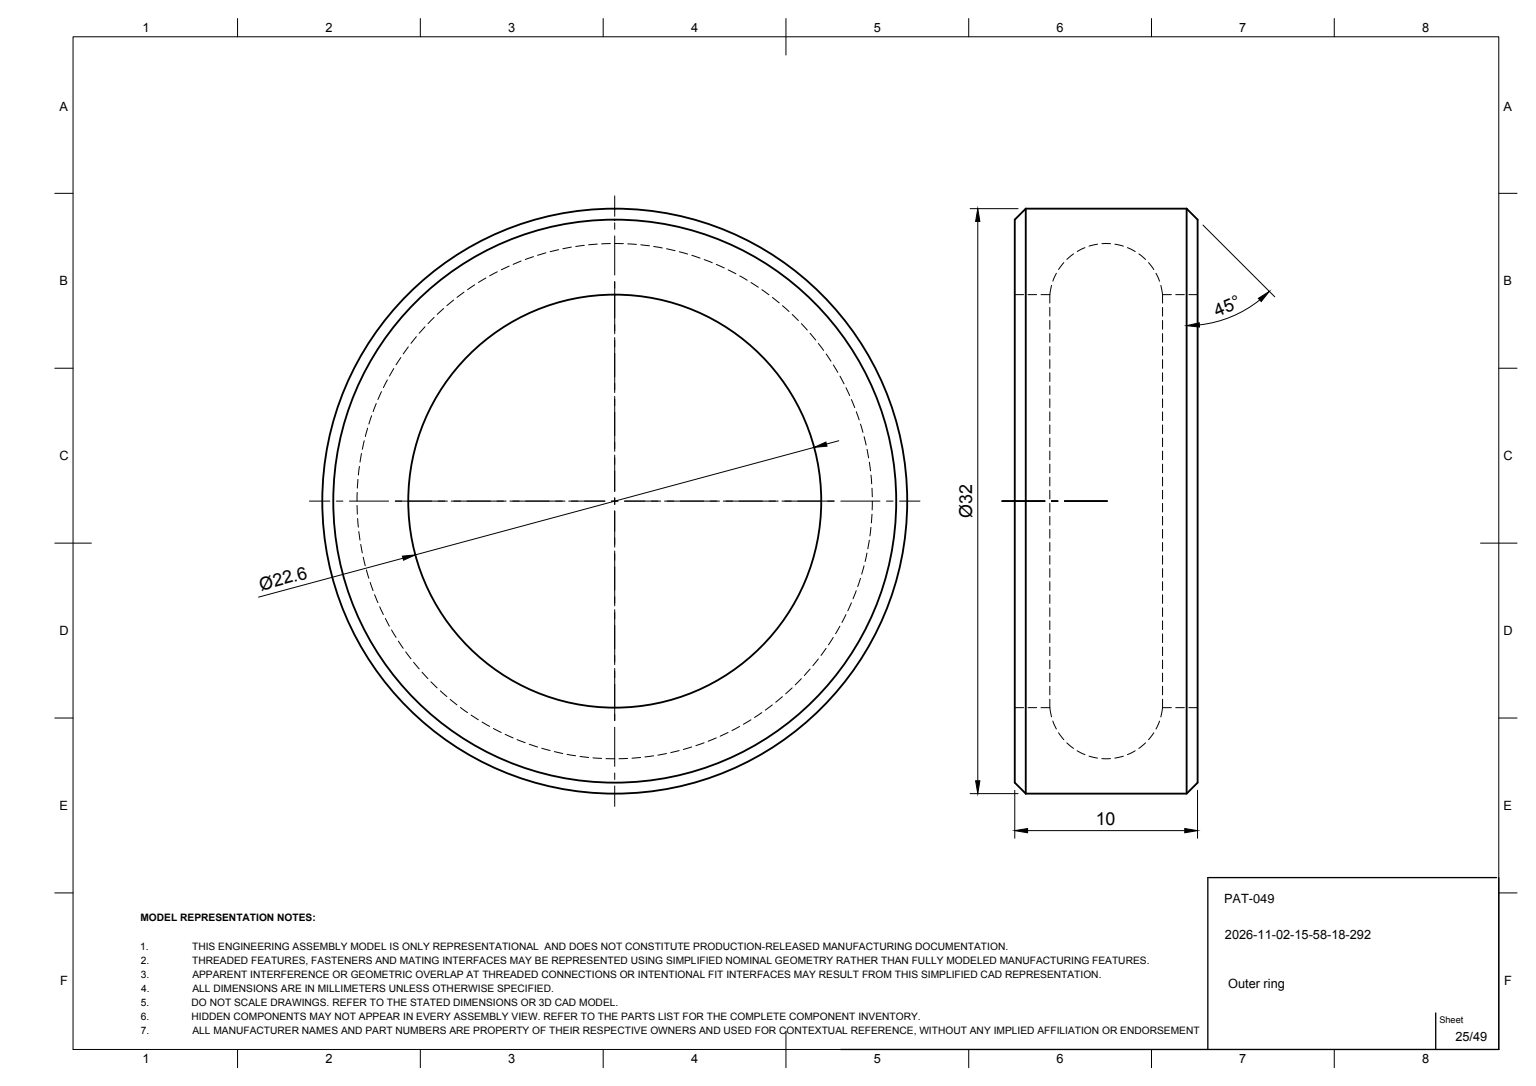
ISO-10303-21;
HEADER;
/* Generated by software containing ST-Developer
 * from STEP Tools, Inc. (www.steptools.com) 
 */

FILE_DESCRIPTION(
/* description */ ('Hand drill press frame (manual)'),
/* implementation_level */ '2;1');

FILE_NAME(
/* name */ 'Outer ring.step',
/* time_stamp */ '2026-10-28T03:25:28-07:00',
/* author */ (''),
/* organization */ (''),
/* preprocessor_version */ 'ST-DEVELOPER v20.2',
/* originating_system */ 'Autodesk Translation Framework v15.17.0.0',
/* authorisation */ '');

FILE_SCHEMA (('AUTOMOTIVE_DESIGN { 1 0 10303 214 3 1 1 }'));
ENDSEC;

DATA;
#10=MECHANICAL_DESIGN_GEOMETRIC_PRESENTATION_REPRESENTATION('',(#637),#33299);
#472=TOROIDAL_SURFACE('',#13625,1.1,0.309556);
#476=CONICAL_SURFACE('',#13636,1.57,0.785398163397449);
#477=CONICAL_SURFACE('',#13640,1.57,0.785398163397449);
#547=SHAPE_REPRESENTATION_RELATIONSHIP('SRR','None',#33507,#592);
#592=ADVANCED_BREP_SHAPE_REPRESENTATION('',(#689),#33269);
#637=STYLED_ITEM('',(#33814),#689);
#689=MANIFOLD_SOLID_BREP('Body1',#12655);
#838=FACE_BOUND('',#2374,.T.);
#839=FACE_BOUND('',#2379,.T.);
#1019=PLANE('',#13633);
#1020=PLANE('',#13642);
#1564=FACE_OUTER_BOUND('',#2371,.T.);
#1565=FACE_OUTER_BOUND('',#2372,.T.);
#1566=FACE_OUTER_BOUND('',#2373,.T.);
#1567=FACE_OUTER_BOUND('',#2375,.T.);
#1568=FACE_OUTER_BOUND('',#2376,.T.);
#1569=FACE_OUTER_BOUND('',#2377,.T.);
#1570=FACE_OUTER_BOUND('',#2378,.T.);
#1571=FACE_OUTER_BOUND('',#2380,.T.);
#2371=EDGE_LOOP('',(#9479,#9480,#9481,#9482,#9483,#9484));
#2372=EDGE_LOOP('',(#9485,#9486,#9487,#9488,#9489));
#2373=EDGE_LOOP('',(#9490));
#2374=EDGE_LOOP('',(#9491));
#2375=EDGE_LOOP('',(#9492,#9493,#9494,#9495));
#2376=EDGE_LOOP('',(#9496,#9497,#9498,#9499));
#2377=EDGE_LOOP('',(#9500,#9501,#9502,#9503));
#2378=EDGE_LOOP('',(#9504));
#2379=EDGE_LOOP('',(#9505));
#2380=EDGE_LOOP('',(#9506,#9507,#9508,#9509,#9510));
#3208=LINE('',#19214,#4373);
#3209=LINE('',#19223,#4374);
#3210=LINE('',#19227,#4375);
#3211=LINE('',#19231,#4376);
#3212=LINE('',#19234,#4377);
#4373=VECTOR('',#15581,1.129765);
#4374=VECTOR('',#15592,1.57);
#4375=VECTOR('',#15597,1.6);
#4376=VECTOR('',#15602,1.57);
#4377=VECTOR('',#15607,1.129765);
#5404=CIRCLE('',#13626,1.129765);
#5405=CIRCLE('',#13627,1.129765);
#5406=CIRCLE('',#13628,0.309556);
#5407=CIRCLE('',#13629,1.129765);
#5408=CIRCLE('',#13630,1.129765);
#5409=CIRCLE('',#13632,1.129765);
#5410=CIRCLE('',#13634,1.54);
#5411=CIRCLE('',#13635,1.129765);
#5412=CIRCLE('',#13637,1.6);
#5413=CIRCLE('',#13639,1.6);
#5414=CIRCLE('',#13641,1.54);
#5965=VERTEX_POINT('',#19202);
#5966=VERTEX_POINT('',#19203);
#5967=VERTEX_POINT('',#19206);
#5968=VERTEX_POINT('',#19208);
#5969=VERTEX_POINT('',#19212);
#5970=VERTEX_POINT('',#19216);
#5971=VERTEX_POINT('',#19218);
#5972=VERTEX_POINT('',#19221);
#5973=VERTEX_POINT('',#19225);
#5974=VERTEX_POINT('',#19229);
#7268=EDGE_CURVE('',#5965,#5966,#5404,.T.);
#7269=EDGE_CURVE('',#5966,#5965,#5405,.T.);
#7270=EDGE_CURVE('',#5966,#5967,#5406,.T.);
#7271=EDGE_CURVE('',#5968,#5967,#5407,.T.);
#7272=EDGE_CURVE('',#5967,#5968,#5408,.T.);
#7273=EDGE_CURVE('',#5969,#5969,#5409,.T.);
#7274=EDGE_CURVE('',#5969,#5968,#3208,.T.);
#7275=EDGE_CURVE('',#5970,#5970,#5410,.T.);
#7276=EDGE_CURVE('',#5971,#5971,#5411,.T.);
#7277=EDGE_CURVE('',#5972,#5972,#5412,.T.);
#7278=EDGE_CURVE('',#5972,#5970,#3209,.T.);
#7279=EDGE_CURVE('',#5973,#5973,#5413,.T.);
#7280=EDGE_CURVE('',#5973,#5972,#3210,.T.);
#7281=EDGE_CURVE('',#5974,#5974,#5414,.T.);
#7282=EDGE_CURVE('',#5974,#5973,#3211,.T.);
#7283=EDGE_CURVE('',#5965,#5971,#3212,.T.);
#9479=ORIENTED_EDGE('',*,*,#7268,.F.);
#9480=ORIENTED_EDGE('',*,*,#7269,.F.);
#9481=ORIENTED_EDGE('',*,*,#7270,.T.);
#9482=ORIENTED_EDGE('',*,*,#7271,.F.);
#9483=ORIENTED_EDGE('',*,*,#7272,.F.);
#9484=ORIENTED_EDGE('',*,*,#7270,.F.);
#9485=ORIENTED_EDGE('',*,*,#7273,.T.);
#9486=ORIENTED_EDGE('',*,*,#7274,.T.);
#9487=ORIENTED_EDGE('',*,*,#7271,.T.);
#9488=ORIENTED_EDGE('',*,*,#7272,.T.);
#9489=ORIENTED_EDGE('',*,*,#7274,.F.);
#9490=ORIENTED_EDGE('',*,*,#7275,.F.);
#9491=ORIENTED_EDGE('',*,*,#7276,.T.);
#9492=ORIENTED_EDGE('',*,*,#7277,.F.);
#9493=ORIENTED_EDGE('',*,*,#7278,.T.);
#9494=ORIENTED_EDGE('',*,*,#7275,.T.);
#9495=ORIENTED_EDGE('',*,*,#7278,.F.);
#9496=ORIENTED_EDGE('',*,*,#7279,.F.);
#9497=ORIENTED_EDGE('',*,*,#7280,.T.);
#9498=ORIENTED_EDGE('',*,*,#7277,.T.);
#9499=ORIENTED_EDGE('',*,*,#7280,.F.);
#9500=ORIENTED_EDGE('',*,*,#7281,.F.);
#9501=ORIENTED_EDGE('',*,*,#7282,.T.);
#9502=ORIENTED_EDGE('',*,*,#7279,.T.);
#9503=ORIENTED_EDGE('',*,*,#7282,.F.);
#9504=ORIENTED_EDGE('',*,*,#7281,.T.);
#9505=ORIENTED_EDGE('',*,*,#7273,.F.);
#9506=ORIENTED_EDGE('',*,*,#7268,.T.);
#9507=ORIENTED_EDGE('',*,*,#7269,.T.);
#9508=ORIENTED_EDGE('',*,*,#7283,.T.);
#9509=ORIENTED_EDGE('',*,*,#7276,.F.);
#9510=ORIENTED_EDGE('',*,*,#7283,.F.);
#11874=CYLINDRICAL_SURFACE('',#13631,1.129765);
#11875=CYLINDRICAL_SURFACE('',#13638,1.6);
#11876=CYLINDRICAL_SURFACE('',#13643,1.129765);
#12173=ADVANCED_FACE('',(#1564),#472,.F.);
#12174=ADVANCED_FACE('',(#1565),#11874,.F.);
#12175=ADVANCED_FACE('',(#1566,#838),#1019,.T.);
#12176=ADVANCED_FACE('',(#1567),#476,.T.);
#12177=ADVANCED_FACE('',(#1568),#11875,.T.);
#12178=ADVANCED_FACE('',(#1569),#477,.T.);
#12179=ADVANCED_FACE('',(#1570,#839),#1020,.T.);
#12180=ADVANCED_FACE('',(#1571),#11876,.F.);
#12655=CLOSED_SHELL('',(#12173,#12174,#12175,#12176,#12177,#12178,#12179,
#12180));
#13624=AXIS2_PLACEMENT_3D('',#19200,#15563,#15564);
#13625=AXIS2_PLACEMENT_3D('',#19201,#15565,#15566);
#13626=AXIS2_PLACEMENT_3D('',#19204,#15567,#15568);
#13627=AXIS2_PLACEMENT_3D('',#19205,#15569,#15570);
#13628=AXIS2_PLACEMENT_3D('',#19207,#15571,#15572);
#13629=AXIS2_PLACEMENT_3D('',#19209,#15573,#15574);
#13630=AXIS2_PLACEMENT_3D('',#19210,#15575,#15576);
#13631=AXIS2_PLACEMENT_3D('',#19211,#15577,#15578);
#13632=AXIS2_PLACEMENT_3D('',#19213,#15579,#15580);
#13633=AXIS2_PLACEMENT_3D('',#19215,#15582,#15583);
#13634=AXIS2_PLACEMENT_3D('',#19217,#15584,#15585);
#13635=AXIS2_PLACEMENT_3D('',#19219,#15586,#15587);
#13636=AXIS2_PLACEMENT_3D('',#19220,#15588,#15589);
#13637=AXIS2_PLACEMENT_3D('',#19222,#15590,#15591);
#13638=AXIS2_PLACEMENT_3D('',#19224,#15593,#15594);
#13639=AXIS2_PLACEMENT_3D('',#19226,#15595,#15596);
#13640=AXIS2_PLACEMENT_3D('',#19228,#15598,#15599);
#13641=AXIS2_PLACEMENT_3D('',#19230,#15600,#15601);
#13642=AXIS2_PLACEMENT_3D('',#19232,#15603,#15604);
#13643=AXIS2_PLACEMENT_3D('',#19233,#15605,#15606);
#15563=DIRECTION('axis',(0.,0.,1.));
#15564=DIRECTION('refdir',(1.,0.,0.));
#15565=DIRECTION('center_axis',(0.,-1.,0.));
#15566=DIRECTION('ref_axis',(0.,0.,-1.));
#15567=DIRECTION('center_axis',(0.,-1.,0.));
#15568=DIRECTION('ref_axis',(1.,0.,0.));
#15569=DIRECTION('center_axis',(0.,-1.,0.));
#15570=DIRECTION('ref_axis',(1.,0.,0.));
#15571=DIRECTION('center_axis',(1.,0.,1.22464679914735E-16));
#15572=DIRECTION('ref_axis',(-1.22464679914735E-16,0.,1.));
#15573=DIRECTION('center_axis',(0.,1.,0.));
#15574=DIRECTION('ref_axis',(1.,0.,0.));
#15575=DIRECTION('center_axis',(0.,1.,0.));
#15576=DIRECTION('ref_axis',(1.,0.,0.));
#15577=DIRECTION('center_axis',(0.,-1.,0.));
#15578=DIRECTION('ref_axis',(1.,0.,0.));
#15579=DIRECTION('center_axis',(0.,-1.,0.));
#15580=DIRECTION('ref_axis',(1.,0.,0.));
#15581=DIRECTION('',(0.,1.,0.));
#15582=DIRECTION('center_axis',(0.,1.,0.));
#15583=DIRECTION('ref_axis',(0.,0.,1.));
#15584=DIRECTION('center_axis',(0.,-1.,0.));
#15585=DIRECTION('ref_axis',(1.,0.,0.));
#15586=DIRECTION('center_axis',(0.,-1.,0.));
#15587=DIRECTION('ref_axis',(1.,0.,0.));
#15588=DIRECTION('center_axis',(0.,-1.,0.));
#15589=DIRECTION('ref_axis',(1.,0.,0.));
#15590=DIRECTION('center_axis',(0.,-1.,0.));
#15591=DIRECTION('ref_axis',(1.,0.,0.));
#15592=DIRECTION('',(0.707106781186548,0.707106781186547,8.65956056235494E-17));
#15593=DIRECTION('center_axis',(0.,-1.,0.));
#15594=DIRECTION('ref_axis',(1.,0.,0.));
#15595=DIRECTION('center_axis',(0.,-1.,0.));
#15596=DIRECTION('ref_axis',(1.,0.,0.));
#15597=DIRECTION('',(0.,1.,0.));
#15598=DIRECTION('center_axis',(0.,1.,0.));
#15599=DIRECTION('ref_axis',(1.,0.,0.));
#15600=DIRECTION('center_axis',(0.,-1.,0.));
#15601=DIRECTION('ref_axis',(1.,0.,0.));
#15602=DIRECTION('',(-0.707106781186548,0.707106781186547,-8.65956056235494E-17));
#15603=DIRECTION('center_axis',(0.,-1.,0.));
#15604=DIRECTION('ref_axis',(0.,0.,-1.));
#15605=DIRECTION('center_axis',(0.,-1.,0.));
#15606=DIRECTION('ref_axis',(1.,0.,0.));
#15607=DIRECTION('',(0.,1.,0.));
#19200=CARTESIAN_POINT('',(0.,0.,0.));
#19201=CARTESIAN_POINT('Origin',(0.,0.,0.));
#19202=CARTESIAN_POINT('',(-1.129765,0.308121667383195,-1.38356309103871E-16));
#19203=CARTESIAN_POINT('',(-1.38356309103871E-16,0.308121667383195,1.129765));
#19204=CARTESIAN_POINT('Origin',(0.,0.308121667383195,0.));
#19205=CARTESIAN_POINT('Origin',(0.,0.308121667383195,0.));
#19206=CARTESIAN_POINT('',(-1.38356309103871E-16,-0.308121667383195,1.129765));
#19207=CARTESIAN_POINT('Origin',(-1.34711147906209E-16,0.,1.1));
#19208=CARTESIAN_POINT('',(-1.129765,-0.308121667383195,1.38356309103871E-16));
#19209=CARTESIAN_POINT('Origin',(0.,-0.308121667383195,0.));
#19210=CARTESIAN_POINT('Origin',(0.,-0.308121667383195,0.));
#19211=CARTESIAN_POINT('Origin',(0.,0.,0.));
#19212=CARTESIAN_POINT('',(-1.129765,-0.5,-1.38356309103871E-16));
#19213=CARTESIAN_POINT('Origin',(0.,-0.5,0.));
#19214=CARTESIAN_POINT('',(-1.129765,0.,-1.38356309103871E-16));
#19215=CARTESIAN_POINT('Origin',(1.54,0.5,0.));
#19216=CARTESIAN_POINT('',(-1.54,0.5,-1.88595607068692E-16));
#19217=CARTESIAN_POINT('Origin',(0.,0.5,0.));
#19218=CARTESIAN_POINT('',(-1.129765,0.5,-1.38356309103871E-16));
#19219=CARTESIAN_POINT('Origin',(0.,0.5,0.));
#19220=CARTESIAN_POINT('Origin',(0.,0.47,0.));
#19221=CARTESIAN_POINT('',(-1.6,0.44,-1.95943487863577E-16));
#19222=CARTESIAN_POINT('Origin',(0.,0.44,0.));
#19223=CARTESIAN_POINT('',(-1.57,0.47,-1.92269547466134E-16));
#19224=CARTESIAN_POINT('Origin',(0.,0.,0.));
#19225=CARTESIAN_POINT('',(-1.6,-0.44,-1.95943487863577E-16));
#19226=CARTESIAN_POINT('Origin',(0.,-0.44,0.));
#19227=CARTESIAN_POINT('',(-1.6,0.,-1.95943487863577E-16));
#19228=CARTESIAN_POINT('Origin',(0.,-0.47,0.));
#19229=CARTESIAN_POINT('',(-1.54,-0.5,-1.88595607068692E-16));
#19230=CARTESIAN_POINT('Origin',(0.,-0.5,0.));
#19231=CARTESIAN_POINT('',(-1.57,-0.47,-1.92269547466134E-16));
#19232=CARTESIAN_POINT('Origin',(1.129765,-0.5,0.));
#19233=CARTESIAN_POINT('Origin',(0.,0.,0.));
#19234=CARTESIAN_POINT('',(-1.129765,0.,-1.38356309103871E-16));
#33217=UNCERTAINTY_MEASURE_WITH_UNIT(LENGTH_MEASURE(0.001),#33300,
'DISTANCE_ACCURACY_VALUE',
'Maximum model space distance between geometric entities at asserted c
onnectivities');
#33247=UNCERTAINTY_MEASURE_WITH_UNIT(LENGTH_MEASURE(0.001),#33300,
'DISTANCE_ACCURACY_VALUE',
'Maximum model space distance between geometric entities at asserted c
onnectivities');
#33269=(
GEOMETRIC_REPRESENTATION_CONTEXT(3)
GLOBAL_UNCERTAINTY_ASSIGNED_CONTEXT((#33217))
GLOBAL_UNIT_ASSIGNED_CONTEXT((#33300,#33302,#33303))
REPRESENTATION_CONTEXT('','3D')
);
#33299=(
GEOMETRIC_REPRESENTATION_CONTEXT(3)
GLOBAL_UNCERTAINTY_ASSIGNED_CONTEXT((#33247))
GLOBAL_UNIT_ASSIGNED_CONTEXT((#33300,#33302,#33303))
REPRESENTATION_CONTEXT('','3D')
);
#33300=(
LENGTH_UNIT()
NAMED_UNIT(*)
SI_UNIT(.CENTI.,.METRE.)
);
#33302=(
NAMED_UNIT(*)
PLANE_ANGLE_UNIT()
SI_UNIT($,.RADIAN.)
);
#33303=(
NAMED_UNIT(*)
SI_UNIT($,.STERADIAN.)
SOLID_ANGLE_UNIT()
);
#33325=SHAPE_DEFINITION_REPRESENTATION(#33376,#33507);
#33376=PRODUCT_DEFINITION_SHAPE('',$,#33559);
#33507=SHAPE_REPRESENTATION('',(#13624),#33269);
#33537=PRODUCT_DEFINITION_CONTEXT('part definition',#33692,'design');
#33559=PRODUCT_DEFINITION('Outer ring','Outer ring',#33610,#33537);
#33610=PRODUCT_DEFINITION_FORMATION('',$,#33715);
#33692=APPLICATION_CONTEXT(
'Core Data for Automotive Mechanical Design Process');
#33693=PRODUCT_CONTEXT('part definition',#33692,'mechanical');
#33715=PRODUCT('Outer ring','Outer ring','Outer ring',(#33693));
#33808=COLOUR_RGB('Grey',0.48,0.52,0.57);
#33809=FILL_AREA_STYLE_COLOUR('',#33808);
#33810=FILL_AREA_STYLE('',(#33809));
#33811=SURFACE_STYLE_FILL_AREA(#33810);
#33812=SURFACE_SIDE_STYLE('',(#33811));
#33813=SURFACE_STYLE_USAGE(.BOTH.,#33812);
#33814=PRESENTATION_STYLE_ASSIGNMENT((#33813));
ENDSEC;
END-ISO-10303-21;
